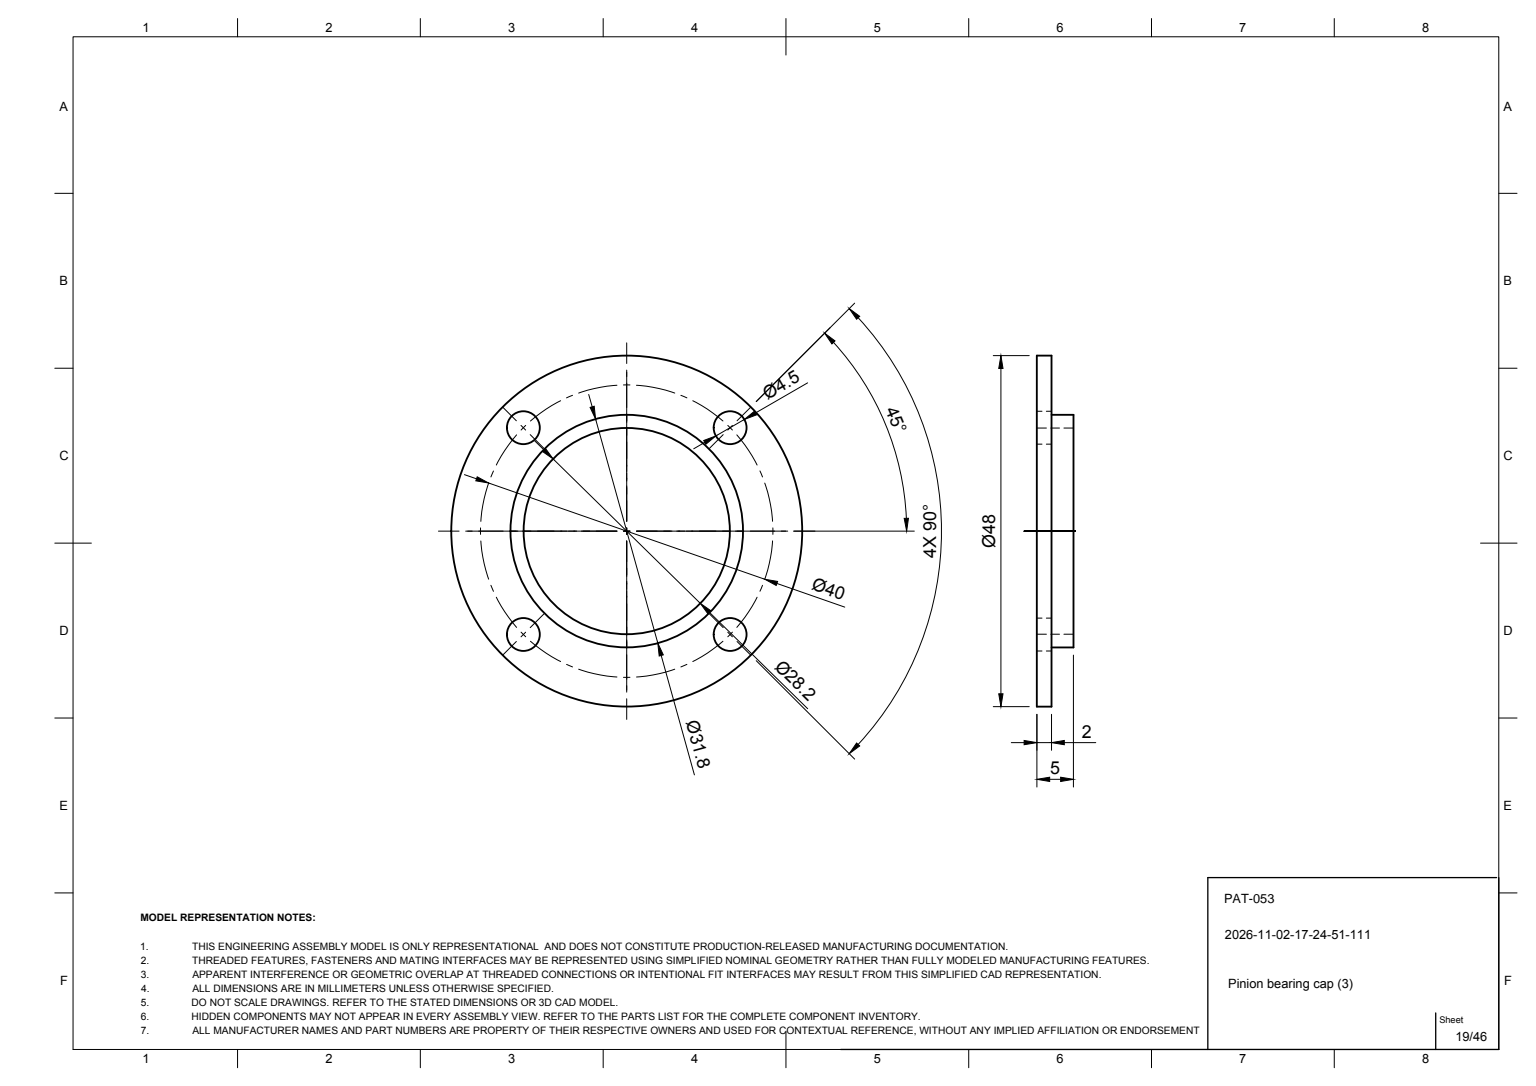
ISO-10303-21;
HEADER;
/* Generated by software containing ST-Developer
 * from STEP Tools, Inc. (www.steptools.com) 
 */

FILE_DESCRIPTION(
/* description */ ('Hand-operated arbor press'),
/* implementation_level */ '2;1');

FILE_NAME(
/* name */ 'Pinion bearing cap (3).step',
/* time_stamp */ '2026-10-28T03:25:25-07:00',
/* author */ (''),
/* organization */ (''),
/* preprocessor_version */ 'ST-DEVELOPER v20.2',
/* originating_system */ 'Autodesk Translation Framework v15.17.0.0',
/* authorisation */ '');

FILE_SCHEMA (('AUTOMOTIVE_DESIGN { 1 0 10303 214 3 1 1 }'));
ENDSEC;

DATA;
#10=MECHANICAL_DESIGN_GEOMETRIC_PRESENTATION_REPRESENTATION('',(#600),#32751);
#516=SHAPE_REPRESENTATION_RELATIONSHIP('SRR','None',#32945,#558);
#558=ADVANCED_BREP_SHAPE_REPRESENTATION('',(#649),#32719);
#600=STYLED_ITEM('',(#33242),#649);
#649=MANIFOLD_SOLID_BREP('Body1',#12497);
#790=FACE_BOUND('',#2283,.T.);
#791=FACE_BOUND('',#2286,.T.);
#792=FACE_BOUND('',#2287,.T.);
#793=FACE_BOUND('',#2288,.T.);
#794=FACE_BOUND('',#2289,.T.);
#795=FACE_BOUND('',#2290,.T.);
#796=FACE_BOUND('',#2292,.T.);
#797=FACE_BOUND('',#2293,.T.);
#798=FACE_BOUND('',#2294,.T.);
#799=FACE_BOUND('',#2295,.T.);
#800=FACE_BOUND('',#2296,.T.);
#963=PLANE('',#13382);
#964=PLANE('',#13386);
#965=PLANE('',#13387);
#1485=FACE_OUTER_BOUND('',#2276,.T.);
#1486=FACE_OUTER_BOUND('',#2277,.T.);
#1487=FACE_OUTER_BOUND('',#2278,.T.);
#1488=FACE_OUTER_BOUND('',#2279,.T.);
#1489=FACE_OUTER_BOUND('',#2280,.T.);
#1490=FACE_OUTER_BOUND('',#2281,.T.);
#1491=FACE_OUTER_BOUND('',#2282,.T.);
#1492=FACE_OUTER_BOUND('',#2284,.T.);
#1493=FACE_OUTER_BOUND('',#2285,.T.);
#1494=FACE_OUTER_BOUND('',#2291,.T.);
#2276=EDGE_LOOP('',(#9236,#9237,#9238,#9239));
#2277=EDGE_LOOP('',(#9240,#9241,#9242,#9243));
#2278=EDGE_LOOP('',(#9244,#9245,#9246,#9247));
#2279=EDGE_LOOP('',(#9248,#9249,#9250,#9251));
#2280=EDGE_LOOP('',(#9252,#9253,#9254,#9255));
#2281=EDGE_LOOP('',(#9256,#9257,#9258,#9259));
#2282=EDGE_LOOP('',(#9260));
#2283=EDGE_LOOP('',(#9261));
#2284=EDGE_LOOP('',(#9262,#9263,#9264,#9265));
#2285=EDGE_LOOP('',(#9266));
#2286=EDGE_LOOP('',(#9267));
#2287=EDGE_LOOP('',(#9268));
#2288=EDGE_LOOP('',(#9269));
#2289=EDGE_LOOP('',(#9270));
#2290=EDGE_LOOP('',(#9271));
#2291=EDGE_LOOP('',(#9272));
#2292=EDGE_LOOP('',(#9273));
#2293=EDGE_LOOP('',(#9274));
#2294=EDGE_LOOP('',(#9275));
#2295=EDGE_LOOP('',(#9276));
#2296=EDGE_LOOP('',(#9277));
#3124=LINE('',#18611,#4295);
#3125=LINE('',#18617,#4296);
#3126=LINE('',#18623,#4297);
#3127=LINE('',#18629,#4298);
#3128=LINE('',#18635,#4299);
#3129=LINE('',#18641,#4300);
#3130=LINE('',#18648,#4301);
#4295=VECTOR('',#15189,1.41);
#4296=VECTOR('',#15196,0.225);
#4297=VECTOR('',#15203,0.225);
#4298=VECTOR('',#15210,0.225);
#4299=VECTOR('',#15217,0.225);
#4300=VECTOR('',#15224,1.59);
#4301=VECTOR('',#15233,2.4);
#5322=CIRCLE('',#13365,1.41);
#5323=CIRCLE('',#13366,1.41);
#5324=CIRCLE('',#13368,0.225);
#5325=CIRCLE('',#13369,0.225);
#5326=CIRCLE('',#13371,0.225);
#5327=CIRCLE('',#13372,0.225);
#5328=CIRCLE('',#13374,0.225);
#5329=CIRCLE('',#13375,0.225);
#5330=CIRCLE('',#13377,0.225);
#5331=CIRCLE('',#13378,0.225);
#5332=CIRCLE('',#13380,1.59);
#5333=CIRCLE('',#13381,1.59);
#5334=CIRCLE('',#13384,2.4);
#5335=CIRCLE('',#13385,2.4);
#5860=VERTEX_POINT('',#18608);
#5861=VERTEX_POINT('',#18610);
#5862=VERTEX_POINT('',#18614);
#5863=VERTEX_POINT('',#18616);
#5864=VERTEX_POINT('',#18620);
#5865=VERTEX_POINT('',#18622);
#5866=VERTEX_POINT('',#18626);
#5867=VERTEX_POINT('',#18628);
#5868=VERTEX_POINT('',#18632);
#5869=VERTEX_POINT('',#18634);
#5870=VERTEX_POINT('',#18638);
#5871=VERTEX_POINT('',#18640);
#5872=VERTEX_POINT('',#18645);
#5873=VERTEX_POINT('',#18647);
#7121=EDGE_CURVE('',#5860,#5860,#5322,.T.);
#7122=EDGE_CURVE('',#5860,#5861,#3124,.T.);
#7123=EDGE_CURVE('',#5861,#5861,#5323,.T.);
#7124=EDGE_CURVE('',#5862,#5862,#5324,.T.);
#7125=EDGE_CURVE('',#5862,#5863,#3125,.T.);
#7126=EDGE_CURVE('',#5863,#5863,#5325,.T.);
#7127=EDGE_CURVE('',#5864,#5864,#5326,.T.);
#7128=EDGE_CURVE('',#5864,#5865,#3126,.T.);
#7129=EDGE_CURVE('',#5865,#5865,#5327,.T.);
#7130=EDGE_CURVE('',#5866,#5866,#5328,.T.);
#7131=EDGE_CURVE('',#5866,#5867,#3127,.T.);
#7132=EDGE_CURVE('',#5867,#5867,#5329,.T.);
#7133=EDGE_CURVE('',#5868,#5868,#5330,.T.);
#7134=EDGE_CURVE('',#5868,#5869,#3128,.T.);
#7135=EDGE_CURVE('',#5869,#5869,#5331,.T.);
#7136=EDGE_CURVE('',#5870,#5870,#5332,.T.);
#7137=EDGE_CURVE('',#5870,#5871,#3129,.T.);
#7138=EDGE_CURVE('',#5871,#5871,#5333,.T.);
#7139=EDGE_CURVE('',#5872,#5872,#5334,.T.);
#7140=EDGE_CURVE('',#5872,#5873,#3130,.T.);
#7141=EDGE_CURVE('',#5873,#5873,#5335,.T.);
#9236=ORIENTED_EDGE('',*,*,#7121,.F.);
#9237=ORIENTED_EDGE('',*,*,#7122,.T.);
#9238=ORIENTED_EDGE('',*,*,#7123,.F.);
#9239=ORIENTED_EDGE('',*,*,#7122,.F.);
#9240=ORIENTED_EDGE('',*,*,#7124,.F.);
#9241=ORIENTED_EDGE('',*,*,#7125,.T.);
#9242=ORIENTED_EDGE('',*,*,#7126,.F.);
#9243=ORIENTED_EDGE('',*,*,#7125,.F.);
#9244=ORIENTED_EDGE('',*,*,#7127,.F.);
#9245=ORIENTED_EDGE('',*,*,#7128,.T.);
#9246=ORIENTED_EDGE('',*,*,#7129,.F.);
#9247=ORIENTED_EDGE('',*,*,#7128,.F.);
#9248=ORIENTED_EDGE('',*,*,#7130,.F.);
#9249=ORIENTED_EDGE('',*,*,#7131,.T.);
#9250=ORIENTED_EDGE('',*,*,#7132,.F.);
#9251=ORIENTED_EDGE('',*,*,#7131,.F.);
#9252=ORIENTED_EDGE('',*,*,#7133,.F.);
#9253=ORIENTED_EDGE('',*,*,#7134,.T.);
#9254=ORIENTED_EDGE('',*,*,#7135,.F.);
#9255=ORIENTED_EDGE('',*,*,#7134,.F.);
#9256=ORIENTED_EDGE('',*,*,#7136,.F.);
#9257=ORIENTED_EDGE('',*,*,#7137,.T.);
#9258=ORIENTED_EDGE('',*,*,#7138,.T.);
#9259=ORIENTED_EDGE('',*,*,#7137,.F.);
#9260=ORIENTED_EDGE('',*,*,#7138,.F.);
#9261=ORIENTED_EDGE('',*,*,#7121,.T.);
#9262=ORIENTED_EDGE('',*,*,#7139,.F.);
#9263=ORIENTED_EDGE('',*,*,#7140,.T.);
#9264=ORIENTED_EDGE('',*,*,#7141,.T.);
#9265=ORIENTED_EDGE('',*,*,#7140,.F.);
#9266=ORIENTED_EDGE('',*,*,#7139,.T.);
#9267=ORIENTED_EDGE('',*,*,#7123,.T.);
#9268=ORIENTED_EDGE('',*,*,#7135,.T.);
#9269=ORIENTED_EDGE('',*,*,#7132,.T.);
#9270=ORIENTED_EDGE('',*,*,#7129,.T.);
#9271=ORIENTED_EDGE('',*,*,#7126,.T.);
#9272=ORIENTED_EDGE('',*,*,#7141,.F.);
#9273=ORIENTED_EDGE('',*,*,#7136,.T.);
#9274=ORIENTED_EDGE('',*,*,#7133,.T.);
#9275=ORIENTED_EDGE('',*,*,#7130,.T.);
#9276=ORIENTED_EDGE('',*,*,#7127,.T.);
#9277=ORIENTED_EDGE('',*,*,#7124,.T.);
#11720=CYLINDRICAL_SURFACE('',#13364,1.41);
#11721=CYLINDRICAL_SURFACE('',#13367,0.225);
#11722=CYLINDRICAL_SURFACE('',#13370,0.225);
#11723=CYLINDRICAL_SURFACE('',#13373,0.225);
#11724=CYLINDRICAL_SURFACE('',#13376,0.225);
#11725=CYLINDRICAL_SURFACE('',#13379,1.59);
#11726=CYLINDRICAL_SURFACE('',#13383,2.4);
#11994=ADVANCED_FACE('',(#1485),#11720,.F.);
#11995=ADVANCED_FACE('',(#1486),#11721,.F.);
#11996=ADVANCED_FACE('',(#1487),#11722,.F.);
#11997=ADVANCED_FACE('',(#1488),#11723,.F.);
#11998=ADVANCED_FACE('',(#1489),#11724,.F.);
#11999=ADVANCED_FACE('',(#1490),#11725,.T.);
#12000=ADVANCED_FACE('',(#1491,#790),#963,.F.);
#12001=ADVANCED_FACE('',(#1492),#11726,.T.);
#12002=ADVANCED_FACE('',(#1493,#791,#792,#793,#794,#795),#964,.T.);
#12003=ADVANCED_FACE('',(#1494,#796,#797,#798,#799,#800),#965,.F.);
#12497=CLOSED_SHELL('',(#11994,#11995,#11996,#11997,#11998,#11999,#12000,
#12001,#12002,#12003));
#13363=AXIS2_PLACEMENT_3D('',#18606,#15183,#15184);
#13364=AXIS2_PLACEMENT_3D('',#18607,#15185,#15186);
#13365=AXIS2_PLACEMENT_3D('',#18609,#15187,#15188);
#13366=AXIS2_PLACEMENT_3D('',#18612,#15190,#15191);
#13367=AXIS2_PLACEMENT_3D('',#18613,#15192,#15193);
#13368=AXIS2_PLACEMENT_3D('',#18615,#15194,#15195);
#13369=AXIS2_PLACEMENT_3D('',#18618,#15197,#15198);
#13370=AXIS2_PLACEMENT_3D('',#18619,#15199,#15200);
#13371=AXIS2_PLACEMENT_3D('',#18621,#15201,#15202);
#13372=AXIS2_PLACEMENT_3D('',#18624,#15204,#15205);
#13373=AXIS2_PLACEMENT_3D('',#18625,#15206,#15207);
#13374=AXIS2_PLACEMENT_3D('',#18627,#15208,#15209);
#13375=AXIS2_PLACEMENT_3D('',#18630,#15211,#15212);
#13376=AXIS2_PLACEMENT_3D('',#18631,#15213,#15214);
#13377=AXIS2_PLACEMENT_3D('',#18633,#15215,#15216);
#13378=AXIS2_PLACEMENT_3D('',#18636,#15218,#15219);
#13379=AXIS2_PLACEMENT_3D('',#18637,#15220,#15221);
#13380=AXIS2_PLACEMENT_3D('',#18639,#15222,#15223);
#13381=AXIS2_PLACEMENT_3D('',#18642,#15225,#15226);
#13382=AXIS2_PLACEMENT_3D('',#18643,#15227,#15228);
#13383=AXIS2_PLACEMENT_3D('',#18644,#15229,#15230);
#13384=AXIS2_PLACEMENT_3D('',#18646,#15231,#15232);
#13385=AXIS2_PLACEMENT_3D('',#18649,#15234,#15235);
#13386=AXIS2_PLACEMENT_3D('',#18650,#15236,#15237);
#13387=AXIS2_PLACEMENT_3D('',#18651,#15238,#15239);
#15183=DIRECTION('axis',(0.,0.,1.));
#15184=DIRECTION('refdir',(1.,0.,0.));
#15185=DIRECTION('center_axis',(0.,1.,0.));
#15186=DIRECTION('ref_axis',(1.,0.,0.));
#15187=DIRECTION('center_axis',(0.,1.,0.));
#15188=DIRECTION('ref_axis',(1.,0.,0.));
#15189=DIRECTION('',(0.,1.,0.));
#15190=DIRECTION('center_axis',(0.,-1.,0.));
#15191=DIRECTION('ref_axis',(1.,0.,0.));
#15192=DIRECTION('center_axis',(0.,1.,0.));
#15193=DIRECTION('ref_axis',(1.,0.,0.));
#15194=DIRECTION('center_axis',(0.,1.,0.));
#15195=DIRECTION('ref_axis',(1.,0.,0.));
#15196=DIRECTION('',(0.,1.,0.));
#15197=DIRECTION('center_axis',(0.,-1.,0.));
#15198=DIRECTION('ref_axis',(1.,0.,0.));
#15199=DIRECTION('center_axis',(0.,1.,0.));
#15200=DIRECTION('ref_axis',(1.,0.,0.));
#15201=DIRECTION('center_axis',(0.,1.,0.));
#15202=DIRECTION('ref_axis',(1.,0.,0.));
#15203=DIRECTION('',(0.,1.,0.));
#15204=DIRECTION('center_axis',(0.,-1.,0.));
#15205=DIRECTION('ref_axis',(1.,0.,0.));
#15206=DIRECTION('center_axis',(0.,1.,0.));
#15207=DIRECTION('ref_axis',(1.,0.,0.));
#15208=DIRECTION('center_axis',(0.,1.,0.));
#15209=DIRECTION('ref_axis',(1.,0.,0.));
#15210=DIRECTION('',(0.,1.,0.));
#15211=DIRECTION('center_axis',(0.,-1.,0.));
#15212=DIRECTION('ref_axis',(1.,0.,0.));
#15213=DIRECTION('center_axis',(0.,1.,0.));
#15214=DIRECTION('ref_axis',(1.,0.,0.));
#15215=DIRECTION('center_axis',(0.,1.,0.));
#15216=DIRECTION('ref_axis',(1.,0.,0.));
#15217=DIRECTION('',(0.,1.,0.));
#15218=DIRECTION('center_axis',(0.,-1.,0.));
#15219=DIRECTION('ref_axis',(1.,0.,0.));
#15220=DIRECTION('center_axis',(0.,1.,0.));
#15221=DIRECTION('ref_axis',(1.,0.,0.));
#15222=DIRECTION('center_axis',(0.,1.,0.));
#15223=DIRECTION('ref_axis',(1.,0.,0.));
#15224=DIRECTION('',(0.,-1.,0.));
#15225=DIRECTION('center_axis',(0.,1.,0.));
#15226=DIRECTION('ref_axis',(1.,0.,0.));
#15227=DIRECTION('center_axis',(0.,1.,0.));
#15228=DIRECTION('ref_axis',(1.,0.,0.));
#15229=DIRECTION('center_axis',(0.,1.,0.));
#15230=DIRECTION('ref_axis',(1.,0.,0.));
#15231=DIRECTION('center_axis',(0.,1.,0.));
#15232=DIRECTION('ref_axis',(1.,0.,0.));
#15233=DIRECTION('',(0.,-1.,0.));
#15234=DIRECTION('center_axis',(0.,1.,0.));
#15235=DIRECTION('ref_axis',(1.,0.,0.));
#15236=DIRECTION('center_axis',(0.,1.,0.));
#15237=DIRECTION('ref_axis',(1.,0.,0.));
#15238=DIRECTION('center_axis',(0.,1.,0.));
#15239=DIRECTION('ref_axis',(1.,0.,0.));
#18606=CARTESIAN_POINT('',(0.,0.,0.));
#18607=CARTESIAN_POINT('Origin',(-3.25,-4.1,20.));
#18608=CARTESIAN_POINT('',(-4.66,3.5,20.));
#18609=CARTESIAN_POINT('Origin',(-3.25,3.5,20.));
#18610=CARTESIAN_POINT('',(-4.66,4.,20.));
#18611=CARTESIAN_POINT('',(-4.66,-4.1,20.));
#18612=CARTESIAN_POINT('Origin',(-3.25,4.,20.));
#18613=CARTESIAN_POINT('Origin',(-4.66421356237309,3.7,18.5857864376269));
#18614=CARTESIAN_POINT('',(-4.88921356237309,3.8,18.5857864376269));
#18615=CARTESIAN_POINT('Origin',(-4.66421356237309,3.8,18.5857864376269));
#18616=CARTESIAN_POINT('',(-4.88921356237309,4.,18.5857864376269));
#18617=CARTESIAN_POINT('',(-4.88921356237309,3.7,18.5857864376269));
#18618=CARTESIAN_POINT('Origin',(-4.66421356237309,4.,18.5857864376269));
#18619=CARTESIAN_POINT('Origin',(-4.66421356237309,3.7,21.4142135623731));
#18620=CARTESIAN_POINT('',(-4.88921356237309,3.8,21.4142135623731));
#18621=CARTESIAN_POINT('Origin',(-4.66421356237309,3.8,21.4142135623731));
#18622=CARTESIAN_POINT('',(-4.88921356237309,4.,21.4142135623731));
#18623=CARTESIAN_POINT('',(-4.88921356237309,3.7,21.4142135623731));
#18624=CARTESIAN_POINT('Origin',(-4.66421356237309,4.,21.4142135623731));
#18625=CARTESIAN_POINT('Origin',(-1.8357864376269,3.7,21.4142135623731));
#18626=CARTESIAN_POINT('',(-2.0607864376269,3.8,21.4142135623731));
#18627=CARTESIAN_POINT('Origin',(-1.8357864376269,3.8,21.4142135623731));
#18628=CARTESIAN_POINT('',(-2.0607864376269,4.,21.4142135623731));
#18629=CARTESIAN_POINT('',(-2.0607864376269,3.7,21.4142135623731));
#18630=CARTESIAN_POINT('Origin',(-1.8357864376269,4.,21.4142135623731));
#18631=CARTESIAN_POINT('Origin',(-1.83578643762691,3.7,18.5857864376269));
#18632=CARTESIAN_POINT('',(-2.06078643762691,3.8,18.5857864376269));
#18633=CARTESIAN_POINT('Origin',(-1.83578643762691,3.8,18.5857864376269));
#18634=CARTESIAN_POINT('',(-2.06078643762691,4.,18.5857864376269));
#18635=CARTESIAN_POINT('',(-2.06078643762691,3.7,18.5857864376269));
#18636=CARTESIAN_POINT('Origin',(-1.83578643762691,4.,18.5857864376269));
#18637=CARTESIAN_POINT('Origin',(-3.25,3.5,20.));
#18638=CARTESIAN_POINT('',(-4.84,3.8,20.));
#18639=CARTESIAN_POINT('Origin',(-3.25,3.8,20.));
#18640=CARTESIAN_POINT('',(-4.84,3.5,20.));
#18641=CARTESIAN_POINT('',(-4.84,3.5,20.));
#18642=CARTESIAN_POINT('Origin',(-3.25,3.5,20.));
#18643=CARTESIAN_POINT('Origin',(-3.25,3.5,20.));
#18644=CARTESIAN_POINT('Origin',(-3.25,3.8,20.));
#18645=CARTESIAN_POINT('',(-5.65,4.,20.));
#18646=CARTESIAN_POINT('Origin',(-3.25,4.,20.));
#18647=CARTESIAN_POINT('',(-5.65,3.8,20.));
#18648=CARTESIAN_POINT('',(-5.65,3.8,20.));
#18649=CARTESIAN_POINT('Origin',(-3.25,3.8,20.));
#18650=CARTESIAN_POINT('Origin',(-3.25,4.,20.));
#18651=CARTESIAN_POINT('Origin',(-3.25,3.8,20.));
#32670=UNCERTAINTY_MEASURE_WITH_UNIT(LENGTH_MEASURE(0.001),#32752,
'DISTANCE_ACCURACY_VALUE',
'Maximum model space distance between geometric entities at asserted c
onnectivities');
#32702=UNCERTAINTY_MEASURE_WITH_UNIT(LENGTH_MEASURE(0.001),#32752,
'DISTANCE_ACCURACY_VALUE',
'Maximum model space distance between geometric entities at asserted c
onnectivities');
#32719=(
GEOMETRIC_REPRESENTATION_CONTEXT(3)
GLOBAL_UNCERTAINTY_ASSIGNED_CONTEXT((#32670))
GLOBAL_UNIT_ASSIGNED_CONTEXT((#32752,#32754,#32755))
REPRESENTATION_CONTEXT('','3D')
);
#32751=(
GEOMETRIC_REPRESENTATION_CONTEXT(3)
GLOBAL_UNCERTAINTY_ASSIGNED_CONTEXT((#32702))
GLOBAL_UNIT_ASSIGNED_CONTEXT((#32752,#32754,#32755))
REPRESENTATION_CONTEXT('','3D')
);
#32752=(
LENGTH_UNIT()
NAMED_UNIT(*)
SI_UNIT(.CENTI.,.METRE.)
);
#32754=(
NAMED_UNIT(*)
PLANE_ANGLE_UNIT()
SI_UNIT($,.RADIAN.)
);
#32755=(
NAMED_UNIT(*)
SI_UNIT($,.STERADIAN.)
SOLID_ANGLE_UNIT()
);
#32772=SHAPE_DEFINITION_REPRESENTATION(#32820,#32945);
#32820=PRODUCT_DEFINITION_SHAPE('',$,#32994);
#32945=SHAPE_REPRESENTATION('',(#13363),#32719);
#32977=PRODUCT_DEFINITION_CONTEXT('part definition',#33123,'design');
#32994=PRODUCT_DEFINITION('Pinion bearing cap (3)',
'Pinion bearing cap (3)',#33042,#32977);
#33042=PRODUCT_DEFINITION_FORMATION('',$,#33141);
#33123=APPLICATION_CONTEXT(
'Core Data for Automotive Mechanical Design Process');
#33124=PRODUCT_CONTEXT('part definition',#33123,'mechanical');
#33141=PRODUCT('Pinion bearing cap (3)','Pinion bearing cap (3)',
'Pinion bearing cap (3)',(#33124));
#33236=COLOUR_RGB('Grey',0.48,0.52,0.57);
#33237=FILL_AREA_STYLE_COLOUR('',#33236);
#33238=FILL_AREA_STYLE('',(#33237));
#33239=SURFACE_STYLE_FILL_AREA(#33238);
#33240=SURFACE_SIDE_STYLE('',(#33239));
#33241=SURFACE_STYLE_USAGE(.BOTH.,#33240);
#33242=PRESENTATION_STYLE_ASSIGNMENT((#33241));
ENDSEC;
END-ISO-10303-21;
